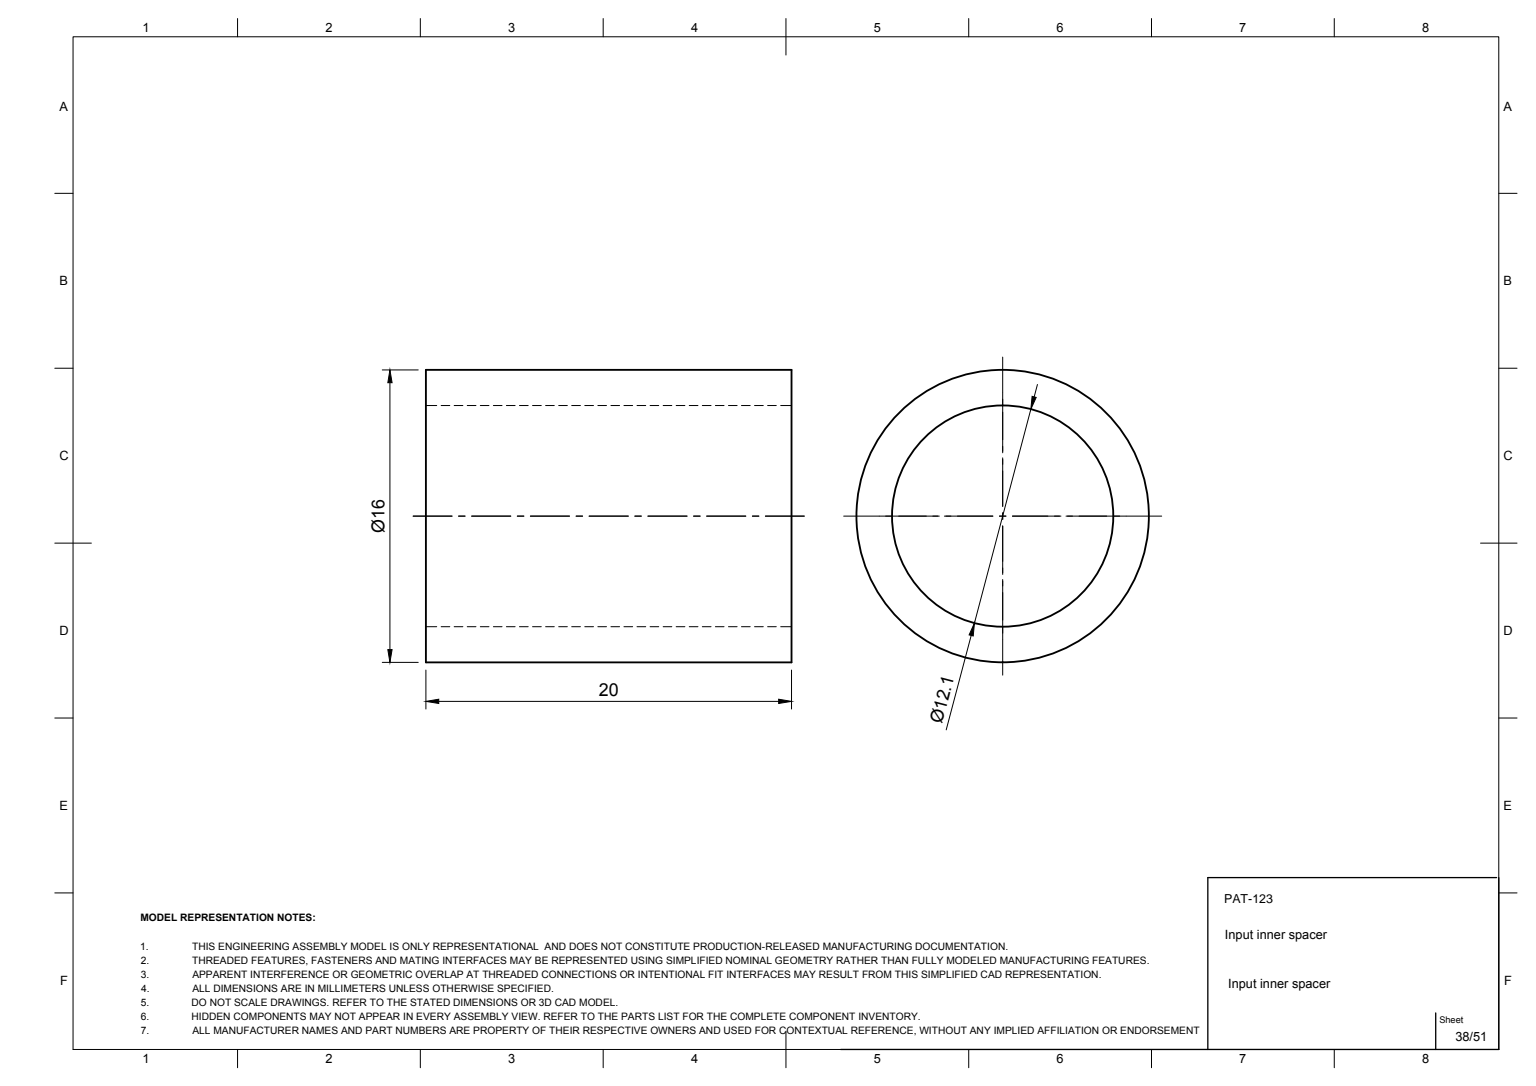
ISO-10303-21;
HEADER;
/* Generated by software containing ST-Developer
 * from STEP Tools, Inc. (www.steptools.com) 
 */

FILE_DESCRIPTION(
/* description */ ('Worm-less right-angle friction wheel drive'),
/* implementation_level */ '2;1');

FILE_NAME(
/* name */ 'Input inner spacer.step',
/* time_stamp */ '2026-10-28T03:22:36-07:00',
/* author */ (''),
/* organization */ (''),
/* preprocessor_version */ 'ST-DEVELOPER v20.2',
/* originating_system */ 'Autodesk Translation Framework v15.17.0.0',
/* authorisation */ '');

FILE_SCHEMA (('AUTOMOTIVE_DESIGN { 1 0 10303 214 3 1 1 }'));
ENDSEC;

DATA;
#10=MECHANICAL_DESIGN_GEOMETRIC_PRESENTATION_REPRESENTATION('',(#651),#17046);
#550=SHAPE_REPRESENTATION_RELATIONSHIP('SRR','None',#17295,#597);
#597=ADVANCED_BREP_SHAPE_REPRESENTATION('',(#702),#17031);
#651=STYLED_ITEM('',(#17605),#702);
#702=MANIFOLD_SOLID_BREP('Body1',#8209);
#923=FACE_BOUND('',#2242,.T.);
#924=FACE_BOUND('',#2244,.T.);
#1135=PLANE('',#9488);
#1136=PLANE('',#9489);
#1565=FACE_OUTER_BOUND('',#2239,.T.);
#1566=FACE_OUTER_BOUND('',#2240,.T.);
#1567=FACE_OUTER_BOUND('',#2241,.T.);
#1568=FACE_OUTER_BOUND('',#2243,.T.);
#2239=EDGE_LOOP('',(#7086,#7087,#7088,#7089));
#2240=EDGE_LOOP('',(#7090,#7091,#7092,#7093));
#2241=EDGE_LOOP('',(#7094));
#2242=EDGE_LOOP('',(#7095));
#2243=EDGE_LOOP('',(#7096));
#2244=EDGE_LOOP('',(#7097));
#2783=LINE('',#16194,#3323);
#2784=LINE('',#16200,#3324);
#3323=VECTOR('',#11663,0.605);
#3324=VECTOR('',#11670,0.8);
#3799=CIRCLE('',#9483,0.605);
#3800=CIRCLE('',#9484,0.605);
#3801=CIRCLE('',#9486,0.8);
#3802=CIRCLE('',#9487,0.8);
#4390=VERTEX_POINT('',#16191);
#4391=VERTEX_POINT('',#16193);
#4392=VERTEX_POINT('',#16197);
#4393=VERTEX_POINT('',#16199);
#5312=EDGE_CURVE('',#4390,#4390,#3799,.T.);
#5313=EDGE_CURVE('',#4390,#4391,#2783,.T.);
#5314=EDGE_CURVE('',#4391,#4391,#3800,.T.);
#5315=EDGE_CURVE('',#4392,#4392,#3801,.T.);
#5316=EDGE_CURVE('',#4392,#4393,#2784,.T.);
#5317=EDGE_CURVE('',#4393,#4393,#3802,.T.);
#7086=ORIENTED_EDGE('',*,*,#5312,.F.);
#7087=ORIENTED_EDGE('',*,*,#5313,.T.);
#7088=ORIENTED_EDGE('',*,*,#5314,.T.);
#7089=ORIENTED_EDGE('',*,*,#5313,.F.);
#7090=ORIENTED_EDGE('',*,*,#5315,.F.);
#7091=ORIENTED_EDGE('',*,*,#5316,.T.);
#7092=ORIENTED_EDGE('',*,*,#5317,.T.);
#7093=ORIENTED_EDGE('',*,*,#5316,.F.);
#7094=ORIENTED_EDGE('',*,*,#5315,.T.);
#7095=ORIENTED_EDGE('',*,*,#5312,.T.);
#7096=ORIENTED_EDGE('',*,*,#5317,.F.);
#7097=ORIENTED_EDGE('',*,*,#5314,.F.);
#7669=CYLINDRICAL_SURFACE('',#9482,0.605);
#7670=CYLINDRICAL_SURFACE('',#9485,0.8);
#8057=ADVANCED_FACE('',(#1565),#7669,.F.);
#8058=ADVANCED_FACE('',(#1566),#7670,.T.);
#8059=ADVANCED_FACE('',(#1567,#923),#1135,.T.);
#8060=ADVANCED_FACE('',(#1568,#924),#1136,.F.);
#8209=CLOSED_SHELL('',(#8057,#8058,#8059,#8060));
#9481=AXIS2_PLACEMENT_3D('',#16189,#11657,#11658);
#9482=AXIS2_PLACEMENT_3D('',#16190,#11659,#11660);
#9483=AXIS2_PLACEMENT_3D('',#16192,#11661,#11662);
#9484=AXIS2_PLACEMENT_3D('',#16195,#11664,#11665);
#9485=AXIS2_PLACEMENT_3D('',#16196,#11666,#11667);
#9486=AXIS2_PLACEMENT_3D('',#16198,#11668,#11669);
#9487=AXIS2_PLACEMENT_3D('',#16201,#11671,#11672);
#9488=AXIS2_PLACEMENT_3D('',#16202,#11673,#11674);
#9489=AXIS2_PLACEMENT_3D('',#16203,#11675,#11676);
#11657=DIRECTION('axis',(0.,0.,1.));
#11658=DIRECTION('refdir',(1.,0.,0.));
#11659=DIRECTION('center_axis',(0.,1.,0.));
#11660=DIRECTION('ref_axis',(1.,0.,0.));
#11661=DIRECTION('center_axis',(0.,-1.,0.));
#11662=DIRECTION('ref_axis',(1.,0.,0.));
#11663=DIRECTION('',(0.,-1.,0.));
#11664=DIRECTION('center_axis',(0.,-1.,0.));
#11665=DIRECTION('ref_axis',(1.,0.,0.));
#11666=DIRECTION('center_axis',(0.,1.,0.));
#11667=DIRECTION('ref_axis',(1.,0.,0.));
#11668=DIRECTION('center_axis',(0.,1.,0.));
#11669=DIRECTION('ref_axis',(1.,0.,0.));
#11670=DIRECTION('',(0.,-1.,0.));
#11671=DIRECTION('center_axis',(0.,1.,0.));
#11672=DIRECTION('ref_axis',(1.,0.,0.));
#11673=DIRECTION('center_axis',(0.,1.,0.));
#11674=DIRECTION('ref_axis',(1.,0.,0.));
#11675=DIRECTION('center_axis',(0.,1.,0.));
#11676=DIRECTION('ref_axis',(1.,0.,0.));
#16189=CARTESIAN_POINT('',(0.,0.,0.));
#16190=CARTESIAN_POINT('Origin',(0.,-6.5,7.));
#16191=CARTESIAN_POINT('',(-0.605,-4.5,7.));
#16192=CARTESIAN_POINT('Origin',(0.,-4.5,7.));
#16193=CARTESIAN_POINT('',(-0.605,-6.5,7.));
#16194=CARTESIAN_POINT('',(-0.605,-6.5,7.));
#16195=CARTESIAN_POINT('Origin',(0.,-6.5,7.));
#16196=CARTESIAN_POINT('Origin',(0.,-6.5,7.));
#16197=CARTESIAN_POINT('',(-0.8,-4.5,7.));
#16198=CARTESIAN_POINT('Origin',(0.,-4.5,7.));
#16199=CARTESIAN_POINT('',(-0.8,-6.5,7.));
#16200=CARTESIAN_POINT('',(-0.8,-6.5,7.));
#16201=CARTESIAN_POINT('Origin',(0.,-6.5,7.));
#16202=CARTESIAN_POINT('Origin',(0.,-4.5,7.));
#16203=CARTESIAN_POINT('Origin',(0.,-6.5,7.));
#16978=UNCERTAINTY_MEASURE_WITH_UNIT(LENGTH_MEASURE(0.001),#17047,
'DISTANCE_ACCURACY_VALUE',
'Maximum model space distance between geometric entities at asserted c
onnectivities');
#16993=UNCERTAINTY_MEASURE_WITH_UNIT(LENGTH_MEASURE(0.001),#17047,
'DISTANCE_ACCURACY_VALUE',
'Maximum model space distance between geometric entities at asserted c
onnectivities');
#17031=(
GEOMETRIC_REPRESENTATION_CONTEXT(3)
GLOBAL_UNCERTAINTY_ASSIGNED_CONTEXT((#16978))
GLOBAL_UNIT_ASSIGNED_CONTEXT((#17047,#17049,#17050))
REPRESENTATION_CONTEXT('','3D')
);
#17046=(
GEOMETRIC_REPRESENTATION_CONTEXT(3)
GLOBAL_UNCERTAINTY_ASSIGNED_CONTEXT((#16993))
GLOBAL_UNIT_ASSIGNED_CONTEXT((#17047,#17049,#17050))
REPRESENTATION_CONTEXT('','3D')
);
#17047=(
LENGTH_UNIT()
NAMED_UNIT(*)
SI_UNIT(.CENTI.,.METRE.)
);
#17049=(
NAMED_UNIT(*)
PLANE_ANGLE_UNIT()
SI_UNIT($,.RADIAN.)
);
#17050=(
NAMED_UNIT(*)
SI_UNIT($,.STERADIAN.)
SOLID_ANGLE_UNIT()
);
#17088=SHAPE_DEFINITION_REPRESENTATION(#17145,#17295);
#17145=PRODUCT_DEFINITION_SHAPE('',$,#17348);
#17295=SHAPE_REPRESENTATION('',(#9481),#17031);
#17310=PRODUCT_DEFINITION_CONTEXT('part definition',#17468,'design');
#17348=PRODUCT_DEFINITION('Input inner spacer','Input inner spacer',#17400,
#17310);
#17400=PRODUCT_DEFINITION_FORMATION('',$,#17507);
#17468=APPLICATION_CONTEXT(
'Core Data for Automotive Mechanical Design Process');
#17469=PRODUCT_CONTEXT('part definition',#17468,'mechanical');
#17507=PRODUCT('Input inner spacer','Input inner spacer',
'Input inner spacer',(#17469));
#17599=COLOUR_RGB('Off White',0.89,0.88,0.83);
#17600=FILL_AREA_STYLE_COLOUR('',#17599);
#17601=FILL_AREA_STYLE('',(#17600));
#17602=SURFACE_STYLE_FILL_AREA(#17601);
#17603=SURFACE_SIDE_STYLE('',(#17602));
#17604=SURFACE_STYLE_USAGE(.BOTH.,#17603);
#17605=PRESENTATION_STYLE_ASSIGNMENT((#17604));
ENDSEC;
END-ISO-10303-21;
